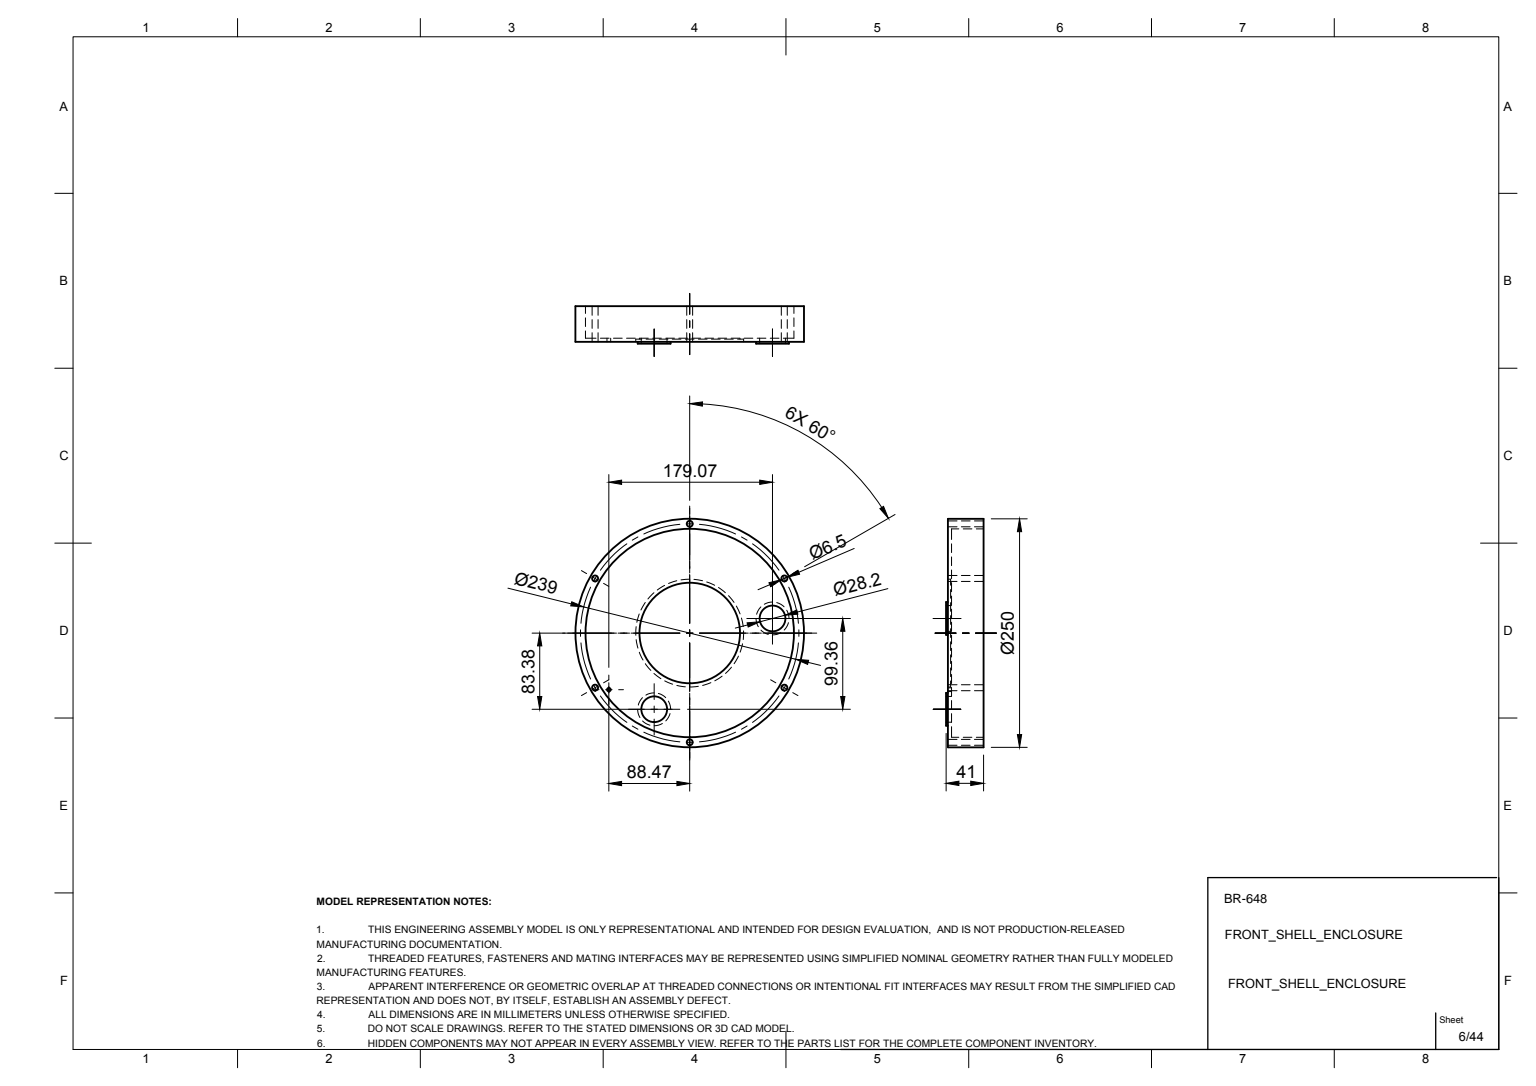
ISO-10303-21;
HEADER;
FILE_DESCRIPTION((''),'2;1');
FILE_NAME('FRONT_SHELL_ENCLOSURE.step','2026-10-01T22:05:39-07:00',(''),(''),'','','');
FILE_SCHEMA (('AUTOMOTIVE_DESIGN { 1 0 10303 214 3 1 1 }'));
ENDSEC;
DATA;
#10=MECHANICAL_DESIGN_GEOMETRIC_PRESENTATION_REPRESENTATION('',(#606),#24628);
#522=SHAPE_REPRESENTATION_RELATIONSHIP('SRR','None',#24794,#564) ;
#564=ADVANCED_BREP_SHAPE_REPRESENTATION('',(#648),#24584) ;
#606=STYLED_ITEM('',(#25031),#648) ;
#648=MANIFOLD_SOLID_BREP('FRONT_SHELL_ENCLOSURE',#13115) ;
#711=FACE_BOUND('',#3795,.T.) ;
#712=FACE_BOUND('',#3799,.T.) ;
#713=FACE_BOUND('',#3802,.T.) ;
#714=FACE_BOUND('',#3806,.T.) ;
#715=FACE_BOUND('',#3807,.T.) ;
#716=FACE_BOUND('',#3808,.T.) ;
#717=FACE_BOUND('',#3809,.T.) ;
#718=FACE_BOUND('',#3812,.T.) ;
#719=FACE_BOUND('',#3813,.T.) ;
#720=FACE_BOUND('',#3814,.T.) ;
#721=FACE_BOUND('',#3815,.T.) ;
#722=FACE_BOUND('',#3816,.T.) ;
#723=FACE_BOUND('',#3817,.T.) ;
#724=FACE_BOUND('',#3818,.T.) ;
#725=FACE_BOUND('',#3820,.T.) ;
#726=FACE_BOUND('',#3821,.T.) ;
#727=FACE_BOUND('',#3822,.T.) ;
#728=FACE_BOUND('',#3823,.T.) ;
#729=FACE_BOUND('',#3824,.T.) ;
#730=FACE_BOUND('',#3825,.T.) ;
#731=FACE_BOUND('',#3826,.T.) ;
#732=FACE_BOUND('',#3827,.T.) ;
#733=FACE_BOUND('',#3828,.T.) ;
#734=FACE_BOUND('',#3829,.T.) ;
#1047=LINE('',#20033,#1883) ;
#1048=LINE('',#20039,#1884) ;
#1049=LINE('',#20045,#1885) ;
#1050=LINE('',#20051,#1886) ;
#1051=LINE('',#20057,#1887) ;
#1052=LINE('',#20063,#1888) ;
#1053=LINE('',#20069,#1889) ;
#1054=LINE('',#20075,#1890) ;
#1055=LINE('',#20081,#1891) ;
#1056=LINE('',#20088,#1892) ;
#1057=LINE('',#20094,#1893) ;
#1058=LINE('',#20101,#1894) ;
#1059=LINE('',#20109,#1895) ;
#1060=LINE('',#20114,#1896) ;
#1061=LINE('',#20121,#1897) ;
#1883=VECTOR('',#15644,0.2025) ;
#1884=VECTOR('',#15651,0.325) ;
#1885=VECTOR('',#15658,0.325) ;
#1886=VECTOR('',#15665,0.325) ;
#1887=VECTOR('',#15672,0.325) ;
#1888=VECTOR('',#15679,0.325) ;
#1889=VECTOR('',#15686,0.325) ;
#1890=VECTOR('',#15693,1.41) ;
#1891=VECTOR('',#15700,1.8) ;
#1892=VECTOR('',#15709,1.41) ;
#1893=VECTOR('',#15716,1.8) ;
#1894=VECTOR('',#15725,5.9) ;
#1895=VECTOR('',#15736,5.5) ;
#1896=VECTOR('',#15741,11.4) ;
#1897=VECTOR('',#15750,12.5) ;
#2693=CYLINDRICAL_SURFACE('',#13754,0.2025) ;
#2694=CYLINDRICAL_SURFACE('',#13757,0.325) ;
#2695=CYLINDRICAL_SURFACE('',#13760,0.325) ;
#2696=CYLINDRICAL_SURFACE('',#13763,0.325) ;
#2697=CYLINDRICAL_SURFACE('',#13766,0.325) ;
#2698=CYLINDRICAL_SURFACE('',#13769,0.325) ;
#2699=CYLINDRICAL_SURFACE('',#13772,0.325) ;
#2700=CYLINDRICAL_SURFACE('',#13775,1.41) ;
#2701=CYLINDRICAL_SURFACE('',#13778,1.8) ;
#2702=CYLINDRICAL_SURFACE('',#13782,1.41) ;
#2703=CYLINDRICAL_SURFACE('',#13785,1.8) ;
#2704=CYLINDRICAL_SURFACE('',#13789,5.9) ;
#2705=CYLINDRICAL_SURFACE('',#13794,5.5) ;
#2706=CYLINDRICAL_SURFACE('',#13796,11.4) ;
#2707=CYLINDRICAL_SURFACE('',#13800,12.5) ;
#2993=FACE_OUTER_BOUND('',#3785,.T.) ;
#2994=FACE_OUTER_BOUND('',#3786,.T.) ;
#2995=FACE_OUTER_BOUND('',#3787,.T.) ;
#2996=FACE_OUTER_BOUND('',#3788,.T.) ;
#2997=FACE_OUTER_BOUND('',#3789,.T.) ;
#2998=FACE_OUTER_BOUND('',#3790,.T.) ;
#2999=FACE_OUTER_BOUND('',#3791,.T.) ;
#3000=FACE_OUTER_BOUND('',#3792,.T.) ;
#3001=FACE_OUTER_BOUND('',#3793,.T.) ;
#3002=FACE_OUTER_BOUND('',#3794,.T.) ;
#3003=FACE_OUTER_BOUND('',#3796,.T.) ;
#3004=FACE_OUTER_BOUND('',#3797,.T.) ;
#3005=FACE_OUTER_BOUND('',#3798,.T.) ;
#3006=FACE_OUTER_BOUND('',#3800,.T.) ;
#3007=FACE_OUTER_BOUND('',#3801,.T.) ;
#3008=FACE_OUTER_BOUND('',#3803,.T.) ;
#3009=FACE_OUTER_BOUND('',#3804,.T.) ;
#3010=FACE_OUTER_BOUND('',#3805,.T.) ;
#3011=FACE_OUTER_BOUND('',#3810,.T.) ;
#3012=FACE_OUTER_BOUND('',#3811,.T.) ;
#3013=FACE_OUTER_BOUND('',#3819,.T.) ;
#3785=EDGE_LOOP('',(#8703,#8704,#8705,#8706)) ;
#3786=EDGE_LOOP('',(#8707,#8708,#8709,#8710)) ;
#3787=EDGE_LOOP('',(#8711,#8712,#8713,#8714)) ;
#3788=EDGE_LOOP('',(#8715,#8716,#8717,#8718)) ;
#3789=EDGE_LOOP('',(#8719,#8720,#8721,#8722)) ;
#3790=EDGE_LOOP('',(#8723,#8724,#8725,#8726)) ;
#3791=EDGE_LOOP('',(#8727,#8728,#8729,#8730)) ;
#3792=EDGE_LOOP('',(#8731,#8732,#8733,#8734)) ;
#3793=EDGE_LOOP('',(#8735,#8736,#8737,#8738)) ;
#3794=EDGE_LOOP('',(#8739)) ;
#3795=EDGE_LOOP('',(#8740)) ;
#3796=EDGE_LOOP('',(#8741,#8742,#8743,#8744)) ;
#3797=EDGE_LOOP('',(#8745,#8746,#8747,#8748)) ;
#3798=EDGE_LOOP('',(#8749)) ;
#3799=EDGE_LOOP('',(#8750)) ;
#3800=EDGE_LOOP('',(#8751,#8752,#8753,#8754)) ;
#3801=EDGE_LOOP('',(#8755)) ;
#3802=EDGE_LOOP('',(#8756)) ;
#3803=EDGE_LOOP('',(#8757,#8758,#8759,#8760)) ;
#3804=EDGE_LOOP('',(#8761,#8762,#8763,#8764)) ;
#3805=EDGE_LOOP('',(#8765)) ;
#3806=EDGE_LOOP('',(#8766)) ;
#3807=EDGE_LOOP('',(#8767)) ;
#3808=EDGE_LOOP('',(#8768)) ;
#3809=EDGE_LOOP('',(#8769)) ;
#3810=EDGE_LOOP('',(#8770,#8771,#8772,#8773)) ;
#3811=EDGE_LOOP('',(#8774)) ;
#3812=EDGE_LOOP('',(#8775)) ;
#3813=EDGE_LOOP('',(#8776)) ;
#3814=EDGE_LOOP('',(#8777)) ;
#3815=EDGE_LOOP('',(#8778)) ;
#3816=EDGE_LOOP('',(#8779)) ;
#3817=EDGE_LOOP('',(#8780)) ;
#3818=EDGE_LOOP('',(#8781)) ;
#3819=EDGE_LOOP('',(#8782)) ;
#3820=EDGE_LOOP('',(#8783)) ;
#3821=EDGE_LOOP('',(#8784)) ;
#3822=EDGE_LOOP('',(#8785)) ;
#3823=EDGE_LOOP('',(#8786)) ;
#3824=EDGE_LOOP('',(#8787)) ;
#3825=EDGE_LOOP('',(#8788)) ;
#3826=EDGE_LOOP('',(#8789)) ;
#3827=EDGE_LOOP('',(#8790)) ;
#3828=EDGE_LOOP('',(#8791)) ;
#3829=EDGE_LOOP('',(#8792)) ;
#4808=CIRCLE('',#13755,0.2025) ;
#4809=CIRCLE('',#13756,0.2025) ;
#4810=CIRCLE('',#13758,0.325) ;
#4811=CIRCLE('',#13759,0.325) ;
#4812=CIRCLE('',#13761,0.325) ;
#4813=CIRCLE('',#13762,0.325) ;
#4814=CIRCLE('',#13764,0.325) ;
#4815=CIRCLE('',#13765,0.325) ;
#4816=CIRCLE('',#13767,0.325) ;
#4817=CIRCLE('',#13768,0.325) ;
#4818=CIRCLE('',#13770,0.325) ;
#4819=CIRCLE('',#13771,0.325) ;
#4820=CIRCLE('',#13773,0.325) ;
#4821=CIRCLE('',#13774,0.325) ;
#4822=CIRCLE('',#13776,1.41) ;
#4823=CIRCLE('',#13777,1.41) ;
#4824=CIRCLE('',#13779,1.8) ;
#4825=CIRCLE('',#13780,1.8) ;
#4826=CIRCLE('',#13783,1.41) ;
#4827=CIRCLE('',#13784,1.41) ;
#4828=CIRCLE('',#13786,1.8) ;
#4829=CIRCLE('',#13787,1.8) ;
#4830=CIRCLE('',#13790,5.9) ;
#4831=CIRCLE('',#13791,5.9) ;
#4832=CIRCLE('',#13793,5.5) ;
#4833=CIRCLE('',#13795,5.5) ;
#4834=CIRCLE('',#13797,11.4) ;
#4835=CIRCLE('',#13798,11.4) ;
#4836=CIRCLE('',#13801,12.5) ;
#4837=CIRCLE('',#13802,12.5) ;
#5609=VERTEX_POINT('',#20030) ;
#5610=VERTEX_POINT('',#20032) ;
#5611=VERTEX_POINT('',#20036) ;
#5612=VERTEX_POINT('',#20038) ;
#5613=VERTEX_POINT('',#20042) ;
#5614=VERTEX_POINT('',#20044) ;
#5615=VERTEX_POINT('',#20048) ;
#5616=VERTEX_POINT('',#20050) ;
#5617=VERTEX_POINT('',#20054) ;
#5618=VERTEX_POINT('',#20056) ;
#5619=VERTEX_POINT('',#20060) ;
#5620=VERTEX_POINT('',#20062) ;
#5621=VERTEX_POINT('',#20066) ;
#5622=VERTEX_POINT('',#20068) ;
#5623=VERTEX_POINT('',#20072) ;
#5624=VERTEX_POINT('',#20074) ;
#5625=VERTEX_POINT('',#20078) ;
#5626=VERTEX_POINT('',#20080) ;
#5627=VERTEX_POINT('',#20085) ;
#5628=VERTEX_POINT('',#20087) ;
#5629=VERTEX_POINT('',#20091) ;
#5630=VERTEX_POINT('',#20093) ;
#5631=VERTEX_POINT('',#20098) ;
#5632=VERTEX_POINT('',#20100) ;
#5633=VERTEX_POINT('',#20104) ;
#5634=VERTEX_POINT('',#20107) ;
#5635=VERTEX_POINT('',#20111) ;
#5636=VERTEX_POINT('',#20113) ;
#5637=VERTEX_POINT('',#20118) ;
#5638=VERTEX_POINT('',#20120) ;
#6841=EDGE_CURVE('',#5609,#5609,#4808,.T.) ;
#6842=EDGE_CURVE('',#5609,#5610,#1047,.T.) ;
#6843=EDGE_CURVE('',#5610,#5610,#4809,.T.) ;
#6844=EDGE_CURVE('',#5611,#5611,#4810,.T.) ;
#6845=EDGE_CURVE('',#5611,#5612,#1048,.T.) ;
#6846=EDGE_CURVE('',#5612,#5612,#4811,.T.) ;
#6847=EDGE_CURVE('',#5613,#5613,#4812,.T.) ;
#6848=EDGE_CURVE('',#5613,#5614,#1049,.T.) ;
#6849=EDGE_CURVE('',#5614,#5614,#4813,.T.) ;
#6850=EDGE_CURVE('',#5615,#5615,#4814,.T.) ;
#6851=EDGE_CURVE('',#5615,#5616,#1050,.T.) ;
#6852=EDGE_CURVE('',#5616,#5616,#4815,.T.) ;
#6853=EDGE_CURVE('',#5617,#5617,#4816,.T.) ;
#6854=EDGE_CURVE('',#5617,#5618,#1051,.T.) ;
#6855=EDGE_CURVE('',#5618,#5618,#4817,.T.) ;
#6856=EDGE_CURVE('',#5619,#5619,#4818,.T.) ;
#6857=EDGE_CURVE('',#5619,#5620,#1052,.T.) ;
#6858=EDGE_CURVE('',#5620,#5620,#4819,.T.) ;
#6859=EDGE_CURVE('',#5621,#5621,#4820,.T.) ;
#6860=EDGE_CURVE('',#5621,#5622,#1053,.T.) ;
#6861=EDGE_CURVE('',#5622,#5622,#4821,.T.) ;
#6862=EDGE_CURVE('',#5623,#5623,#4822,.T.) ;
#6863=EDGE_CURVE('',#5623,#5624,#1054,.T.) ;
#6864=EDGE_CURVE('',#5624,#5624,#4823,.T.) ;
#6865=EDGE_CURVE('',#5625,#5625,#4824,.T.) ;
#6866=EDGE_CURVE('',#5625,#5626,#1055,.T.) ;
#6867=EDGE_CURVE('',#5626,#5626,#4825,.T.) ;
#6868=EDGE_CURVE('',#5627,#5627,#4826,.T.) ;
#6869=EDGE_CURVE('',#5627,#5628,#1056,.T.) ;
#6870=EDGE_CURVE('',#5628,#5628,#4827,.T.) ;
#6871=EDGE_CURVE('',#5629,#5629,#4828,.T.) ;
#6872=EDGE_CURVE('',#5629,#5630,#1057,.T.) ;
#6873=EDGE_CURVE('',#5630,#5630,#4829,.T.) ;
#6874=EDGE_CURVE('',#5631,#5631,#4830,.T.) ;
#6875=EDGE_CURVE('',#5631,#5632,#1058,.T.) ;
#6876=EDGE_CURVE('',#5632,#5632,#4831,.T.) ;
#6877=EDGE_CURVE('',#5633,#5633,#4832,.T.) ;
#6878=EDGE_CURVE('',#5634,#5634,#4833,.T.) ;
#6879=EDGE_CURVE('',#5634,#5633,#1059,.T.) ;
#6880=EDGE_CURVE('',#5635,#5635,#4834,.T.) ;
#6881=EDGE_CURVE('',#5635,#5636,#1060,.T.) ;
#6882=EDGE_CURVE('',#5636,#5636,#4835,.T.) ;
#6883=EDGE_CURVE('',#5637,#5637,#4836,.T.) ;
#6884=EDGE_CURVE('',#5637,#5638,#1061,.T.) ;
#6885=EDGE_CURVE('',#5638,#5638,#4837,.T.) ;
#8703=ORIENTED_EDGE('',*,*,#6841,.F.) ;
#8704=ORIENTED_EDGE('',*,*,#6842,.T.) ;
#8705=ORIENTED_EDGE('',*,*,#6843,.F.) ;
#8706=ORIENTED_EDGE('',*,*,#6842,.F.) ;
#8707=ORIENTED_EDGE('',*,*,#6844,.F.) ;
#8708=ORIENTED_EDGE('',*,*,#6845,.T.) ;
#8709=ORIENTED_EDGE('',*,*,#6846,.F.) ;
#8710=ORIENTED_EDGE('',*,*,#6845,.F.) ;
#8711=ORIENTED_EDGE('',*,*,#6847,.F.) ;
#8712=ORIENTED_EDGE('',*,*,#6848,.T.) ;
#8713=ORIENTED_EDGE('',*,*,#6849,.F.) ;
#8714=ORIENTED_EDGE('',*,*,#6848,.F.) ;
#8715=ORIENTED_EDGE('',*,*,#6850,.F.) ;
#8716=ORIENTED_EDGE('',*,*,#6851,.T.) ;
#8717=ORIENTED_EDGE('',*,*,#6852,.F.) ;
#8718=ORIENTED_EDGE('',*,*,#6851,.F.) ;
#8719=ORIENTED_EDGE('',*,*,#6853,.F.) ;
#8720=ORIENTED_EDGE('',*,*,#6854,.T.) ;
#8721=ORIENTED_EDGE('',*,*,#6855,.F.) ;
#8722=ORIENTED_EDGE('',*,*,#6854,.F.) ;
#8723=ORIENTED_EDGE('',*,*,#6856,.F.) ;
#8724=ORIENTED_EDGE('',*,*,#6857,.T.) ;
#8725=ORIENTED_EDGE('',*,*,#6858,.F.) ;
#8726=ORIENTED_EDGE('',*,*,#6857,.F.) ;
#8727=ORIENTED_EDGE('',*,*,#6859,.F.) ;
#8728=ORIENTED_EDGE('',*,*,#6860,.T.) ;
#8729=ORIENTED_EDGE('',*,*,#6861,.F.) ;
#8730=ORIENTED_EDGE('',*,*,#6860,.F.) ;
#8731=ORIENTED_EDGE('',*,*,#6862,.F.) ;
#8732=ORIENTED_EDGE('',*,*,#6863,.T.) ;
#8733=ORIENTED_EDGE('',*,*,#6864,.F.) ;
#8734=ORIENTED_EDGE('',*,*,#6863,.F.) ;
#8735=ORIENTED_EDGE('',*,*,#6865,.F.) ;
#8736=ORIENTED_EDGE('',*,*,#6866,.T.) ;
#8737=ORIENTED_EDGE('',*,*,#6867,.F.) ;
#8738=ORIENTED_EDGE('',*,*,#6866,.F.) ;
#8739=ORIENTED_EDGE('',*,*,#6865,.T.) ;
#8740=ORIENTED_EDGE('',*,*,#6864,.T.) ;
#8741=ORIENTED_EDGE('',*,*,#6868,.F.) ;
#8742=ORIENTED_EDGE('',*,*,#6869,.T.) ;
#8743=ORIENTED_EDGE('',*,*,#6870,.F.) ;
#8744=ORIENTED_EDGE('',*,*,#6869,.F.) ;
#8745=ORIENTED_EDGE('',*,*,#6871,.F.) ;
#8746=ORIENTED_EDGE('',*,*,#6872,.T.) ;
#8747=ORIENTED_EDGE('',*,*,#6873,.F.) ;
#8748=ORIENTED_EDGE('',*,*,#6872,.F.) ;
#8749=ORIENTED_EDGE('',*,*,#6871,.T.) ;
#8750=ORIENTED_EDGE('',*,*,#6870,.T.) ;
#8751=ORIENTED_EDGE('',*,*,#6874,.T.) ;
#8752=ORIENTED_EDGE('',*,*,#6875,.T.) ;
#8753=ORIENTED_EDGE('',*,*,#6876,.F.) ;
#8754=ORIENTED_EDGE('',*,*,#6875,.F.) ;
#8755=ORIENTED_EDGE('',*,*,#6874,.F.) ;
#8756=ORIENTED_EDGE('',*,*,#6877,.F.) ;
#8757=ORIENTED_EDGE('',*,*,#6878,.F.) ;
#8758=ORIENTED_EDGE('',*,*,#6879,.T.) ;
#8759=ORIENTED_EDGE('',*,*,#6877,.T.) ;
#8760=ORIENTED_EDGE('',*,*,#6879,.F.) ;
#8761=ORIENTED_EDGE('',*,*,#6880,.F.) ;
#8762=ORIENTED_EDGE('',*,*,#6881,.T.) ;
#8763=ORIENTED_EDGE('',*,*,#6882,.T.) ;
#8764=ORIENTED_EDGE('',*,*,#6881,.F.) ;
#8765=ORIENTED_EDGE('',*,*,#6882,.F.) ;
#8766=ORIENTED_EDGE('',*,*,#6841,.T.) ;
#8767=ORIENTED_EDGE('',*,*,#6862,.T.) ;
#8768=ORIENTED_EDGE('',*,*,#6868,.T.) ;
#8769=ORIENTED_EDGE('',*,*,#6878,.T.) ;
#8770=ORIENTED_EDGE('',*,*,#6883,.F.) ;
#8771=ORIENTED_EDGE('',*,*,#6884,.T.) ;
#8772=ORIENTED_EDGE('',*,*,#6885,.F.) ;
#8773=ORIENTED_EDGE('',*,*,#6884,.F.) ;
#8774=ORIENTED_EDGE('',*,*,#6885,.T.) ;
#8775=ORIENTED_EDGE('',*,*,#6844,.T.) ;
#8776=ORIENTED_EDGE('',*,*,#6847,.T.) ;
#8777=ORIENTED_EDGE('',*,*,#6850,.T.) ;
#8778=ORIENTED_EDGE('',*,*,#6853,.T.) ;
#8779=ORIENTED_EDGE('',*,*,#6856,.T.) ;
#8780=ORIENTED_EDGE('',*,*,#6859,.T.) ;
#8781=ORIENTED_EDGE('',*,*,#6880,.T.) ;
#8782=ORIENTED_EDGE('',*,*,#6883,.T.) ;
#8783=ORIENTED_EDGE('',*,*,#6846,.T.) ;
#8784=ORIENTED_EDGE('',*,*,#6876,.T.) ;
#8785=ORIENTED_EDGE('',*,*,#6873,.T.) ;
#8786=ORIENTED_EDGE('',*,*,#6867,.T.) ;
#8787=ORIENTED_EDGE('',*,*,#6861,.T.) ;
#8788=ORIENTED_EDGE('',*,*,#6858,.T.) ;
#8789=ORIENTED_EDGE('',*,*,#6855,.T.) ;
#8790=ORIENTED_EDGE('',*,*,#6852,.T.) ;
#8791=ORIENTED_EDGE('',*,*,#6849,.T.) ;
#8792=ORIENTED_EDGE('',*,*,#6843,.T.) ;
#12016=PLANE('',#13781) ;
#12017=PLANE('',#13788) ;
#12018=PLANE('',#13792) ;
#12019=PLANE('',#13799) ;
#12020=PLANE('',#13803) ;
#12021=PLANE('',#13804) ;
#12388=ADVANCED_FACE('',(#2993),#2693,.F.) ;
#12389=ADVANCED_FACE('',(#2994),#2694,.F.) ;
#12390=ADVANCED_FACE('',(#2995),#2695,.F.) ;
#12391=ADVANCED_FACE('',(#2996),#2696,.F.) ;
#12392=ADVANCED_FACE('',(#2997),#2697,.F.) ;
#12393=ADVANCED_FACE('',(#2998),#2698,.F.) ;
#12394=ADVANCED_FACE('',(#2999),#2699,.F.) ;
#12395=ADVANCED_FACE('',(#3000),#2700,.F.) ;
#12396=ADVANCED_FACE('',(#3001),#2701,.T.) ;
#12397=ADVANCED_FACE('',(#3002,#711),#12016,.T.) ;
#12398=ADVANCED_FACE('',(#3003),#2702,.F.) ;
#12399=ADVANCED_FACE('',(#3004),#2703,.T.) ;
#12400=ADVANCED_FACE('',(#3005,#712),#12017,.T.) ;
#12401=ADVANCED_FACE('',(#3006),#2704,.F.) ;
#12402=ADVANCED_FACE('',(#3007,#713),#12018,.F.) ;
#12403=ADVANCED_FACE('',(#3008),#2705,.F.) ;
#12404=ADVANCED_FACE('',(#3009),#2706,.F.) ;
#12405=ADVANCED_FACE('',(#3010,#714,#715,#716,#717),#12019,.F.) ;
#12406=ADVANCED_FACE('',(#3011),#2707,.T.) ;
#12407=ADVANCED_FACE('',(#3012,#718,#719,#720,#721,#722,#723,#724),#12020,
 .T.) ;
#12408=ADVANCED_FACE('',(#3013,#725,#726,#727,#728,#729,#730,#731,#732,
#733,#734),#12021,.T.) ;
#13115=CLOSED_SHELL('',(#12388,#12389,#12390,#12391,#12392,#12393,#12394,
#12395,#12396,#12397,#12398,#12399,#12400,#12401,#12402,#12403,#12404,#12405,
#12406,#12407,#12408)) ;
#13753=AXIS2_PLACEMENT_3D('',#20028,#15638,#15639) ;
#13754=AXIS2_PLACEMENT_3D('',#20029,#15640,#15641) ;
#13755=AXIS2_PLACEMENT_3D('',#20031,#15642,#15643) ;
#13756=AXIS2_PLACEMENT_3D('',#20034,#15645,#15646) ;
#13757=AXIS2_PLACEMENT_3D('',#20035,#15647,#15648) ;
#13758=AXIS2_PLACEMENT_3D('',#20037,#15649,#15650) ;
#13759=AXIS2_PLACEMENT_3D('',#20040,#15652,#15653) ;
#13760=AXIS2_PLACEMENT_3D('',#20041,#15654,#15655) ;
#13761=AXIS2_PLACEMENT_3D('',#20043,#15656,#15657) ;
#13762=AXIS2_PLACEMENT_3D('',#20046,#15659,#15660) ;
#13763=AXIS2_PLACEMENT_3D('',#20047,#15661,#15662) ;
#13764=AXIS2_PLACEMENT_3D('',#20049,#15663,#15664) ;
#13765=AXIS2_PLACEMENT_3D('',#20052,#15666,#15667) ;
#13766=AXIS2_PLACEMENT_3D('',#20053,#15668,#15669) ;
#13767=AXIS2_PLACEMENT_3D('',#20055,#15670,#15671) ;
#13768=AXIS2_PLACEMENT_3D('',#20058,#15673,#15674) ;
#13769=AXIS2_PLACEMENT_3D('',#20059,#15675,#15676) ;
#13770=AXIS2_PLACEMENT_3D('',#20061,#15677,#15678) ;
#13771=AXIS2_PLACEMENT_3D('',#20064,#15680,#15681) ;
#13772=AXIS2_PLACEMENT_3D('',#20065,#15682,#15683) ;
#13773=AXIS2_PLACEMENT_3D('',#20067,#15684,#15685) ;
#13774=AXIS2_PLACEMENT_3D('',#20070,#15687,#15688) ;
#13775=AXIS2_PLACEMENT_3D('',#20071,#15689,#15690) ;
#13776=AXIS2_PLACEMENT_3D('',#20073,#15691,#15692) ;
#13777=AXIS2_PLACEMENT_3D('',#20076,#15694,#15695) ;
#13778=AXIS2_PLACEMENT_3D('',#20077,#15696,#15697) ;
#13779=AXIS2_PLACEMENT_3D('',#20079,#15698,#15699) ;
#13780=AXIS2_PLACEMENT_3D('',#20082,#15701,#15702) ;
#13781=AXIS2_PLACEMENT_3D('',#20083,#15703,#15704) ;
#13782=AXIS2_PLACEMENT_3D('',#20084,#15705,#15706) ;
#13783=AXIS2_PLACEMENT_3D('',#20086,#15707,#15708) ;
#13784=AXIS2_PLACEMENT_3D('',#20089,#15710,#15711) ;
#13785=AXIS2_PLACEMENT_3D('',#20090,#15712,#15713) ;
#13786=AXIS2_PLACEMENT_3D('',#20092,#15714,#15715) ;
#13787=AXIS2_PLACEMENT_3D('',#20095,#15717,#15718) ;
#13788=AXIS2_PLACEMENT_3D('',#20096,#15719,#15720) ;
#13789=AXIS2_PLACEMENT_3D('',#20097,#15721,#15722) ;
#13790=AXIS2_PLACEMENT_3D('',#20099,#15723,#15724) ;
#13791=AXIS2_PLACEMENT_3D('',#20102,#15726,#15727) ;
#13792=AXIS2_PLACEMENT_3D('',#20103,#15728,#15729) ;
#13793=AXIS2_PLACEMENT_3D('',#20105,#15730,#15731) ;
#13794=AXIS2_PLACEMENT_3D('',#20106,#15732,#15733) ;
#13795=AXIS2_PLACEMENT_3D('',#20108,#15734,#15735) ;
#13796=AXIS2_PLACEMENT_3D('',#20110,#15737,#15738) ;
#13797=AXIS2_PLACEMENT_3D('',#20112,#15739,#15740) ;
#13798=AXIS2_PLACEMENT_3D('',#20115,#15742,#15743) ;
#13799=AXIS2_PLACEMENT_3D('',#20116,#15744,#15745) ;
#13800=AXIS2_PLACEMENT_3D('',#20117,#15746,#15747) ;
#13801=AXIS2_PLACEMENT_3D('',#20119,#15748,#15749) ;
#13802=AXIS2_PLACEMENT_3D('',#20122,#15751,#15752) ;
#13803=AXIS2_PLACEMENT_3D('',#20123,#15753,#15754) ;
#13804=AXIS2_PLACEMENT_3D('',#20124,#15755,#15756) ;
#15638=DIRECTION('axis',(0.,0.,1.)) ;
#15639=DIRECTION('refdir',(1.,0.,0.)) ;
#15640=DIRECTION('center_axis',(0.,1.,0.)) ;
#15641=DIRECTION('ref_axis',(1.,0.,0.)) ;
#15642=DIRECTION('center_axis',(0.,1.,0.)) ;
#15643=DIRECTION('ref_axis',(1.,0.,0.)) ;
#15644=DIRECTION('',(0.,1.,0.)) ;
#15645=DIRECTION('center_axis',(0.,-1.,0.)) ;
#15646=DIRECTION('ref_axis',(1.,0.,0.)) ;
#15647=DIRECTION('center_axis',(0.,1.,0.)) ;
#15648=DIRECTION('ref_axis',(1.,0.,0.)) ;
#15649=DIRECTION('center_axis',(0.,1.,0.)) ;
#15650=DIRECTION('ref_axis',(1.,0.,0.)) ;
#15651=DIRECTION('',(0.,1.,0.)) ;
#15652=DIRECTION('center_axis',(0.,-1.,0.)) ;
#15653=DIRECTION('ref_axis',(1.,0.,0.)) ;
#15654=DIRECTION('center_axis',(0.,1.,0.)) ;
#15655=DIRECTION('ref_axis',(1.,0.,0.)) ;
#15656=DIRECTION('center_axis',(0.,1.,0.)) ;
#15657=DIRECTION('ref_axis',(1.,0.,0.)) ;
#15658=DIRECTION('',(0.,1.,0.)) ;
#15659=DIRECTION('center_axis',(0.,-1.,0.)) ;
#15660=DIRECTION('ref_axis',(1.,0.,0.)) ;
#15661=DIRECTION('center_axis',(0.,1.,0.)) ;
#15662=DIRECTION('ref_axis',(1.,0.,0.)) ;
#15663=DIRECTION('center_axis',(0.,1.,0.)) ;
#15664=DIRECTION('ref_axis',(1.,0.,0.)) ;
#15665=DIRECTION('',(0.,1.,0.)) ;
#15666=DIRECTION('center_axis',(0.,-1.,0.)) ;
#15667=DIRECTION('ref_axis',(1.,0.,0.)) ;
#15668=DIRECTION('center_axis',(0.,1.,0.)) ;
#15669=DIRECTION('ref_axis',(1.,0.,0.)) ;
#15670=DIRECTION('center_axis',(0.,1.,0.)) ;
#15671=DIRECTION('ref_axis',(1.,0.,0.)) ;
#15672=DIRECTION('',(0.,1.,0.)) ;
#15673=DIRECTION('center_axis',(0.,-1.,0.)) ;
#15674=DIRECTION('ref_axis',(1.,0.,0.)) ;
#15675=DIRECTION('center_axis',(0.,1.,0.)) ;
#15676=DIRECTION('ref_axis',(1.,0.,0.)) ;
#15677=DIRECTION('center_axis',(0.,1.,0.)) ;
#15678=DIRECTION('ref_axis',(1.,0.,0.)) ;
#15679=DIRECTION('',(0.,1.,0.)) ;
#15680=DIRECTION('center_axis',(0.,-1.,0.)) ;
#15681=DIRECTION('ref_axis',(1.,0.,0.)) ;
#15682=DIRECTION('center_axis',(0.,1.,0.)) ;
#15683=DIRECTION('ref_axis',(1.,0.,0.)) ;
#15684=DIRECTION('center_axis',(0.,1.,0.)) ;
#15685=DIRECTION('ref_axis',(1.,0.,0.)) ;
#15686=DIRECTION('',(0.,1.,0.)) ;
#15687=DIRECTION('center_axis',(0.,-1.,0.)) ;
#15688=DIRECTION('ref_axis',(1.,0.,0.)) ;
#15689=DIRECTION('center_axis',(0.,1.,0.)) ;
#15690=DIRECTION('ref_axis',(1.,0.,0.)) ;
#15691=DIRECTION('center_axis',(0.,1.,0.)) ;
#15692=DIRECTION('ref_axis',(1.,0.,0.)) ;
#15693=DIRECTION('',(0.,1.,0.)) ;
#15694=DIRECTION('center_axis',(0.,-1.,0.)) ;
#15695=DIRECTION('ref_axis',(1.,0.,0.)) ;
#15696=DIRECTION('center_axis',(0.,1.,0.)) ;
#15697=DIRECTION('ref_axis',(1.,0.,0.)) ;
#15698=DIRECTION('center_axis',(0.,1.,0.)) ;
#15699=DIRECTION('ref_axis',(1.,0.,0.)) ;
#15700=DIRECTION('',(0.,-1.,0.)) ;
#15701=DIRECTION('center_axis',(0.,-1.,0.)) ;
#15702=DIRECTION('ref_axis',(1.,0.,0.)) ;
#15703=DIRECTION('center_axis',(0.,1.,0.)) ;
#15704=DIRECTION('ref_axis',(1.,0.,0.)) ;
#15705=DIRECTION('center_axis',(0.,1.,0.)) ;
#15706=DIRECTION('ref_axis',(1.,0.,0.)) ;
#15707=DIRECTION('center_axis',(0.,1.,0.)) ;
#15708=DIRECTION('ref_axis',(1.,0.,0.)) ;
#15709=DIRECTION('',(0.,1.,0.)) ;
#15710=DIRECTION('center_axis',(0.,-1.,0.)) ;
#15711=DIRECTION('ref_axis',(1.,0.,0.)) ;
#15712=DIRECTION('center_axis',(0.,1.,0.)) ;
#15713=DIRECTION('ref_axis',(1.,0.,0.)) ;
#15714=DIRECTION('center_axis',(0.,1.,0.)) ;
#15715=DIRECTION('ref_axis',(1.,0.,0.)) ;
#15716=DIRECTION('',(0.,-1.,0.)) ;
#15717=DIRECTION('center_axis',(0.,-1.,0.)) ;
#15718=DIRECTION('ref_axis',(1.,0.,0.)) ;
#15719=DIRECTION('center_axis',(0.,1.,0.)) ;
#15720=DIRECTION('ref_axis',(1.,0.,0.)) ;
#15721=DIRECTION('center_axis',(0.,1.,0.)) ;
#15722=DIRECTION('ref_axis',(1.,0.,0.)) ;
#15723=DIRECTION('center_axis',(0.,-1.,0.)) ;
#15724=DIRECTION('ref_axis',(1.,0.,0.)) ;
#15725=DIRECTION('',(0.,1.,0.)) ;
#15726=DIRECTION('center_axis',(0.,-1.,0.)) ;
#15727=DIRECTION('ref_axis',(1.,0.,0.)) ;
#15728=DIRECTION('center_axis',(0.,-1.,0.)) ;
#15729=DIRECTION('ref_axis',(-1.,0.,0.)) ;
#15730=DIRECTION('center_axis',(0.,1.,0.)) ;
#15731=DIRECTION('ref_axis',(1.,0.,0.)) ;
#15732=DIRECTION('center_axis',(0.,1.,0.)) ;
#15733=DIRECTION('ref_axis',(1.,0.,0.)) ;
#15734=DIRECTION('center_axis',(0.,1.,0.)) ;
#15735=DIRECTION('ref_axis',(1.,0.,0.)) ;
#15736=DIRECTION('',(0.,1.,0.)) ;
#15737=DIRECTION('center_axis',(0.,1.,0.)) ;
#15738=DIRECTION('ref_axis',(1.,0.,0.)) ;
#15739=DIRECTION('center_axis',(0.,1.,0.)) ;
#15740=DIRECTION('ref_axis',(1.,0.,0.)) ;
#15741=DIRECTION('',(0.,1.,0.)) ;
#15742=DIRECTION('center_axis',(0.,1.,0.)) ;
#15743=DIRECTION('ref_axis',(1.,0.,0.)) ;
#15744=DIRECTION('center_axis',(0.,1.,0.)) ;
#15745=DIRECTION('ref_axis',(1.,0.,0.)) ;
#15746=DIRECTION('center_axis',(0.,1.,0.)) ;
#15747=DIRECTION('ref_axis',(1.,0.,0.)) ;
#15748=DIRECTION('center_axis',(0.,1.,0.)) ;
#15749=DIRECTION('ref_axis',(1.,0.,0.)) ;
#15750=DIRECTION('',(0.,-1.,0.)) ;
#15751=DIRECTION('center_axis',(0.,-1.,0.)) ;
#15752=DIRECTION('ref_axis',(1.,0.,0.)) ;
#15753=DIRECTION('center_axis',(0.,-1.,0.)) ;
#15754=DIRECTION('ref_axis',(-1.,0.,0.)) ;
#15755=DIRECTION('center_axis',(0.,1.,0.)) ;
#15756=DIRECTION('ref_axis',(1.,0.,0.)) ;
#20028=CARTESIAN_POINT('',(0.,0.,0.)) ;
#20029=CARTESIAN_POINT('Origin',(-6.1946255125913,3.75,8.84684207832111)) ;
#20030=CARTESIAN_POINT('',(-6.3971255125913,3.6,8.84684207832111)) ;
#20031=CARTESIAN_POINT('Origin',(-6.1946255125913,3.6,8.84684207832111)) ;
#20032=CARTESIAN_POINT('',(-6.3971255125913,4.,8.84684207832111)) ;
#20033=CARTESIAN_POINT('',(-6.3971255125913,3.75,8.84684207832111)) ;
#20034=CARTESIAN_POINT('Origin',(-6.1946255125913,4.,8.84684207832111)) ;
#20035=CARTESIAN_POINT('Origin',(5.975,2.,-10.349003575224)) ;
#20036=CARTESIAN_POINT('',(5.65,0.0999999999999999,-10.349003575224)) ;
#20037=CARTESIAN_POINT('Origin',(5.975,0.0999999999999999,-10.349003575224)) ;
#20038=CARTESIAN_POINT('',(5.65,4.,-10.349003575224)) ;
#20039=CARTESIAN_POINT('',(5.65,2.,-10.349003575224)) ;
#20040=CARTESIAN_POINT('Origin',(5.975,4.,-10.349003575224)) ;
#20041=CARTESIAN_POINT('Origin',(-5.975,2.,-10.349003575224)) ;
#20042=CARTESIAN_POINT('',(-6.30000000000001,0.0999999999999999,-10.349003575224)) ;
#20043=CARTESIAN_POINT('Origin',(-5.975,0.0999999999999999,-10.349003575224)) ;
#20044=CARTESIAN_POINT('',(-6.30000000000001,4.,-10.349003575224)) ;
#20045=CARTESIAN_POINT('',(-6.30000000000001,2.,-10.349003575224)) ;
#20046=CARTESIAN_POINT('Origin',(-5.975,4.,-10.349003575224)) ;
#20047=CARTESIAN_POINT('Origin',(-11.95,2.,1.46345292498109E-15)) ;
#20048=CARTESIAN_POINT('',(-12.275,0.0999999999999999,1.50325394595338E-15)) ;
#20049=CARTESIAN_POINT('Origin',(-11.95,0.0999999999999999,1.46345292498109E-15)) ;
#20050=CARTESIAN_POINT('',(-12.275,4.,1.4236519040088E-15)) ;
#20051=CARTESIAN_POINT('',(-12.275,2.,1.50325394595338E-15)) ;
#20052=CARTESIAN_POINT('Origin',(-11.95,4.,1.46345292498109E-15)) ;
#20053=CARTESIAN_POINT('Origin',(-5.975,2.,10.349003575224)) ;
#20054=CARTESIAN_POINT('',(-6.3,0.0999999999999999,10.349003575224)) ;
#20055=CARTESIAN_POINT('Origin',(-5.975,0.0999999999999999,10.349003575224)) ;
#20056=CARTESIAN_POINT('',(-6.3,4.,10.349003575224)) ;
#20057=CARTESIAN_POINT('',(-6.3,2.,10.349003575224)) ;
#20058=CARTESIAN_POINT('Origin',(-5.975,4.,10.349003575224)) ;
#20059=CARTESIAN_POINT('Origin',(5.975,2.,10.349003575224)) ;
#20060=CARTESIAN_POINT('',(5.65,0.0999999999999999,10.349003575224)) ;
#20061=CARTESIAN_POINT('Origin',(5.975,0.0999999999999999,10.349003575224)) ;
#20062=CARTESIAN_POINT('',(5.65,4.,10.349003575224)) ;
#20063=CARTESIAN_POINT('',(5.65,2.,10.349003575224)) ;
#20064=CARTESIAN_POINT('Origin',(5.975,4.,10.349003575224)) ;
#20065=CARTESIAN_POINT('Origin',(11.95,2.,0.)) ;
#20066=CARTESIAN_POINT('',(11.625,0.0999999999999999,3.9801020972289E-17)) ;
#20067=CARTESIAN_POINT('Origin',(11.95,0.0999999999999999,0.)) ;
#20068=CARTESIAN_POINT('',(11.625,4.,-3.9801020972289E-17)) ;
#20069=CARTESIAN_POINT('',(11.625,2.,3.9801020972289E-17)) ;
#20070=CARTESIAN_POINT('Origin',(11.95,4.,0.)) ;
#20071=CARTESIAN_POINT('Origin',(1.59756323453576,3.65,-9.06023132771231)) ;
#20072=CARTESIAN_POINT('',(0.187563234535756,3.6,-9.06023132771231)) ;
#20073=CARTESIAN_POINT('Origin',(1.59756323453576,3.6,-9.06023132771231)) ;
#20074=CARTESIAN_POINT('',(0.187563234535756,4.2,-9.06023132771231)) ;
#20075=CARTESIAN_POINT('',(0.187563234535756,3.65,-9.06023132771231)) ;
#20076=CARTESIAN_POINT('Origin',(1.59756323453576,4.2,-9.06023132771231)) ;
#20077=CARTESIAN_POINT('Origin',(1.59756323453576,3.9,-9.06023132771231)) ;
#20078=CARTESIAN_POINT('',(-0.202436765464244,4.2,-9.06023132771231)) ;
#20079=CARTESIAN_POINT('Origin',(1.59756323453576,4.2,-9.06023132771231)) ;
#20080=CARTESIAN_POINT('',(-0.202436765464244,4.,-9.06023132771231)) ;
#20081=CARTESIAN_POINT('',(-0.202436765464244,3.9,-9.06023132771231)) ;
#20082=CARTESIAN_POINT('Origin',(1.59756323453576,4.,-9.06023132771231)) ;
#20083=CARTESIAN_POINT('Origin',(1.59756323453576,4.2,-9.06023132771231)) ;
#20084=CARTESIAN_POINT('Origin',(-8.33803164073718,3.65,3.88808800801444)) ;
#20085=CARTESIAN_POINT('',(-9.74803164073718,3.6,3.88808800801444)) ;
#20086=CARTESIAN_POINT('Origin',(-8.33803164073718,3.6,3.88808800801444)) ;
#20087=CARTESIAN_POINT('',(-9.74803164073718,4.2,3.88808800801444)) ;
#20088=CARTESIAN_POINT('',(-9.74803164073718,3.65,3.88808800801444)) ;
#20089=CARTESIAN_POINT('Origin',(-8.33803164073718,4.2,3.88808800801444)) ;
#20090=CARTESIAN_POINT('Origin',(-8.33803164073718,3.9,3.88808800801444)) ;
#20091=CARTESIAN_POINT('',(-10.1380316407372,4.2,3.88808800801444)) ;
#20092=CARTESIAN_POINT('Origin',(-8.33803164073718,4.2,3.88808800801444)) ;
#20093=CARTESIAN_POINT('',(-10.1380316407372,4.,3.88808800801444)) ;
#20094=CARTESIAN_POINT('',(-10.1380316407372,3.9,3.88808800801444)) ;
#20095=CARTESIAN_POINT('Origin',(-8.33803164073718,4.,3.88808800801444)) ;
#20096=CARTESIAN_POINT('Origin',(-8.33803164073718,4.2,3.88808800801444)) ;
#20097=CARTESIAN_POINT('Origin',(0.,3.9,0.)) ;
#20098=CARTESIAN_POINT('',(-5.9,3.7,7.22541611496938E-16)) ;
#20099=CARTESIAN_POINT('Origin',(0.,3.7,0.)) ;
#20100=CARTESIAN_POINT('',(-5.9,4.,-7.22541611496938E-16)) ;
#20101=CARTESIAN_POINT('',(-5.9,3.9,7.22541611496938E-16)) ;
#20102=CARTESIAN_POINT('Origin',(0.,4.,0.)) ;
#20103=CARTESIAN_POINT('Origin',(0.,3.7,0.)) ;
#20104=CARTESIAN_POINT('',(-5.5,3.7,6.73555739531044E-16)) ;
#20105=CARTESIAN_POINT('Origin',(0.,3.7,0.)) ;
#20106=CARTESIAN_POINT('Origin',(0.,3.8,0.)) ;
#20107=CARTESIAN_POINT('',(-5.5,3.6,6.73555739531044E-16)) ;
#20108=CARTESIAN_POINT('Origin',(0.,3.6,0.)) ;
#20109=CARTESIAN_POINT('',(-5.5,3.8,6.73555739531044E-16)) ;
#20110=CARTESIAN_POINT('Origin',(0.,1.8,0.)) ;
#20111=CARTESIAN_POINT('',(-11.4,0.0999999999999999,1.39609735102798E-15)) ;
#20112=CARTESIAN_POINT('Origin',(0.,0.0999999999999999,0.)) ;
#20113=CARTESIAN_POINT('',(-11.4,3.6,1.39609735102798E-15)) ;
#20114=CARTESIAN_POINT('',(-11.4,1.8,1.39609735102798E-15)) ;
#20115=CARTESIAN_POINT('Origin',(0.,3.6,0.)) ;
#20116=CARTESIAN_POINT('Origin',(0.,3.6,0.)) ;
#20117=CARTESIAN_POINT('Origin',(0.,2.05,0.)) ;
#20118=CARTESIAN_POINT('',(-12.5,4.,1.53080849893419E-15)) ;
#20119=CARTESIAN_POINT('Origin',(0.,4.,0.)) ;
#20120=CARTESIAN_POINT('',(-12.5,0.0999999999999999,1.53080849893419E-15)) ;
#20121=CARTESIAN_POINT('',(-12.5,2.05,1.53080849893419E-15)) ;
#20122=CARTESIAN_POINT('Origin',(0.,0.0999999999999999,0.)) ;
#20123=CARTESIAN_POINT('Origin',(0.,0.0999999999999999,0.)) ;
#20124=CARTESIAN_POINT('Origin',(0.,4.,0.)) ;
#24536=UNCERTAINTY_MEASURE_WITH_UNIT(LENGTH_MEASURE(0.001),#24629,
'DISTANCE_ACCURACY_VALUE',
'Maximum model space distance between geometric entities at asserted c
onnectivities') ;
#24580=UNCERTAINTY_MEASURE_WITH_UNIT(LENGTH_MEASURE(0.001),#24629,
'DISTANCE_ACCURACY_VALUE',
'Maximum model space distance between geometric entities at asserted c
onnectivities') ;
#24584=(
GEOMETRIC_REPRESENTATION_CONTEXT(3)
GLOBAL_UNCERTAINTY_ASSIGNED_CONTEXT((#24536))
GLOBAL_UNIT_ASSIGNED_CONTEXT((#24629,#24631,#24632))
REPRESENTATION_CONTEXT('','3D')
) ;
#24628=(
GEOMETRIC_REPRESENTATION_CONTEXT(3)
GLOBAL_UNCERTAINTY_ASSIGNED_CONTEXT((#24580))
GLOBAL_UNIT_ASSIGNED_CONTEXT((#24629,#24631,#24632))
REPRESENTATION_CONTEXT('','3D')
) ;
#24629=(
LENGTH_UNIT()
NAMED_UNIT(*)
SI_UNIT(.CENTI.,.METRE.)
) ;
#24631=(
NAMED_UNIT(*)
PLANE_ANGLE_UNIT()
SI_UNIT($,.RADIAN.)
) ;
#24632=(
NAMED_UNIT(*)
SI_UNIT($,.STERADIAN.)
SOLID_ANGLE_UNIT()
) ;
#24636=SHAPE_DEFINITION_REPRESENTATION(#24683,#24794) ;
#24683=PRODUCT_DEFINITION_SHAPE('',$,#24842) ;
#24794=SHAPE_REPRESENTATION('',(#13753),#24584) ;
#24838=PRODUCT_DEFINITION_CONTEXT('part definition',#24981,'design') ;
#24842=PRODUCT_DEFINITION('FRONT_SHELL_ENCLOSURE',
'FRONT_SHELL_ENCLOSURE',#24889,#24838) ;
#24889=PRODUCT_DEFINITION_FORMATION('',$,#24986) ;
#24981=APPLICATION_CONTEXT(
'Core Data for Automotive Mechanical Design Process') ;
#24982=PRODUCT_CONTEXT('part definition',#24981,'mechanical') ;
#24986=PRODUCT('FRONT_SHELL_ENCLOSURE','FRONT_SHELL_ENCLOSURE',$,(#24982)) ;
#25031=PRESENTATION_STYLE_ASSIGNMENT((#25041)) ;
#25041=SURFACE_STYLE_USAGE(.BOTH.,#25051) ;
#25051=SURFACE_SIDE_STYLE('',(#25061)) ;
#25061=SURFACE_STYLE_FILL_AREA(#25071) ;
#25071=FILL_AREA_STYLE('Aluminum - Satin',(#25081)) ;
#25081=FILL_AREA_STYLE_COLOUR('Aluminum - Satin',#25091) ;
#25091=COLOUR_RGB('Aluminum - Satin', 0.40784314, 0.44705882, 0.49803922) ;
ENDSEC;
END-ISO-10303-21;
